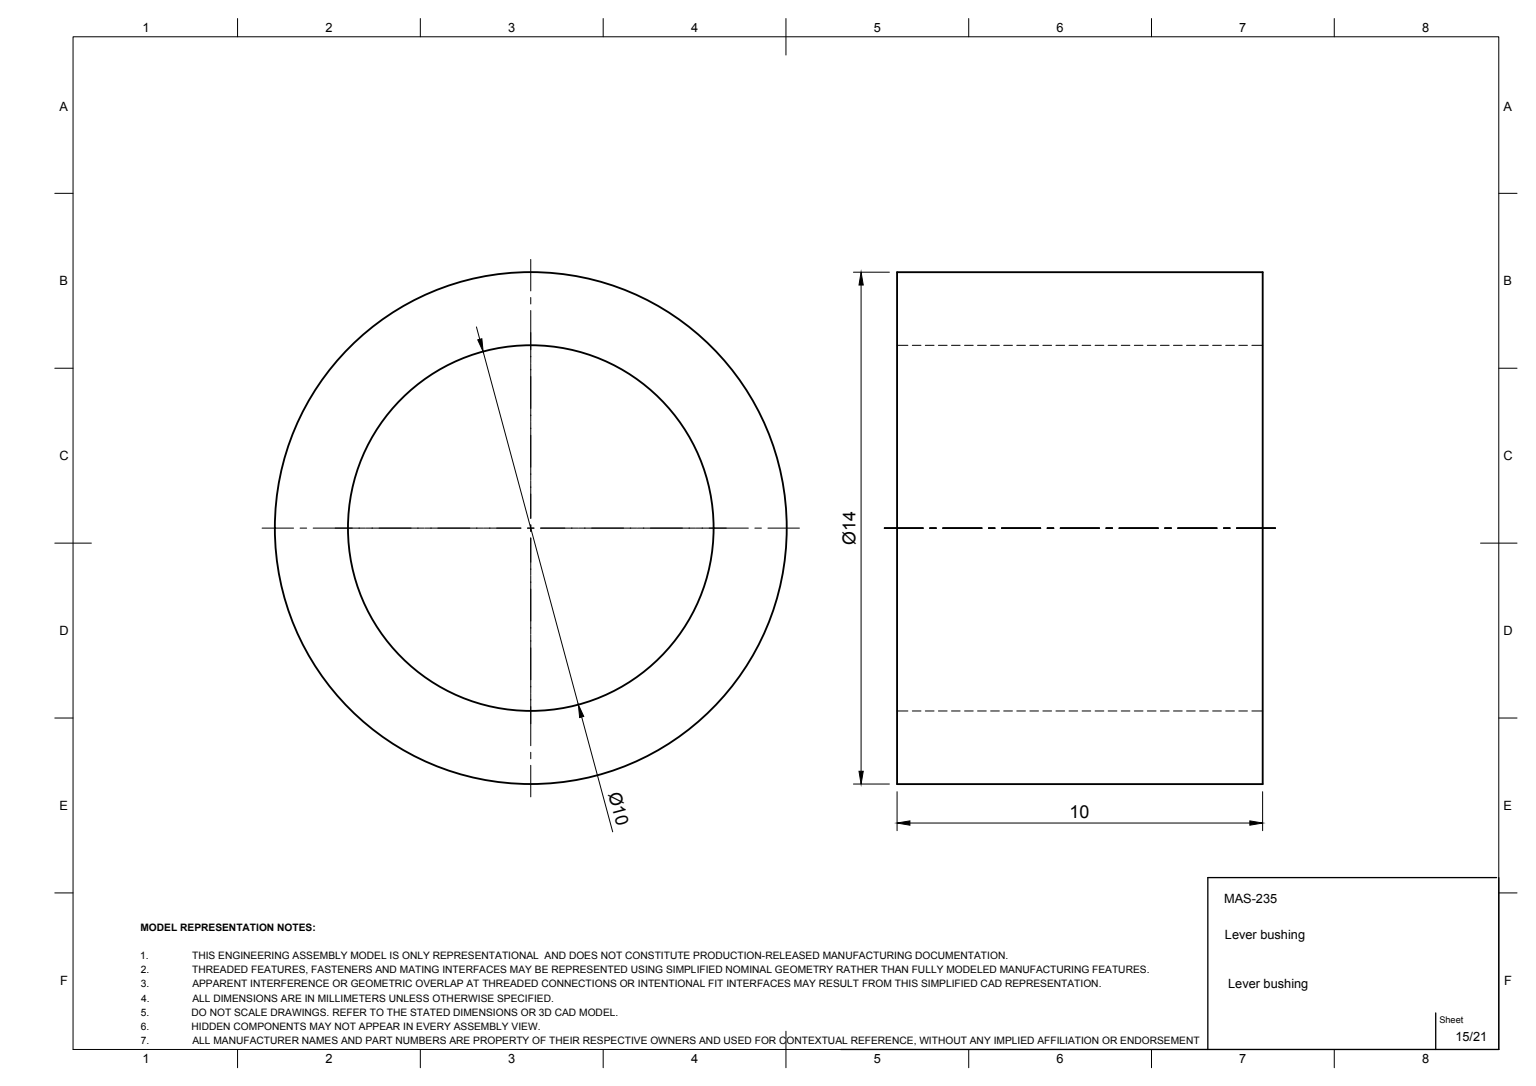
ISO-10303-21;
HEADER;
/* Generated by software containing ST-Developer
 * from STEP Tools, Inc. (www.steptools.com) 
 */

FILE_DESCRIPTION(
/* description */ ('Independent Whitworth quick-return mechanism. Crank radius40, ground-
center spacing80, lever180, connecting rod160, output guide X200. Nomi
nal stroke180 and long/short phase ratio2. Retained guide rods, replac
eable bearing sleeves and captured sliding shoe. No load or production
 rating assigned.'),
/* implementation_level */ '2;1');

FILE_NAME(
/* name */ 'Lever bushing.step',
/* time_stamp */ '2026-11-09T18:22:56-08:00',
/* author */ (''),
/* organization */ (''),
/* preprocessor_version */ 'ST-DEVELOPER v20.2',
/* originating_system */ 'Autodesk Translation Framework v15.17.0.0',
/* authorisation */ '');

FILE_SCHEMA (('AUTOMOTIVE_DESIGN { 1 0 10303 214 3 1 1 }'));
ENDSEC;

DATA;
#10=MECHANICAL_DESIGN_GEOMETRIC_PRESENTATION_REPRESENTATION('',(#236),#4388);
#196=SHAPE_REPRESENTATION_RELATIONSHIP('SRR','None',#4495,#216);
#216=ADVANCED_BREP_SHAPE_REPRESENTATION('',(#256),#4385);
#236=STYLED_ITEM('',(#4597),#256);
#256=MANIFOLD_SOLID_BREP('Body1',#2341);
#315=FACE_BOUND('',#744,.T.);
#316=FACE_BOUND('',#746,.T.);
#397=PLANE('',#2833);
#398=PLANE('',#2834);
#538=FACE_OUTER_BOUND('',#741,.T.);
#539=FACE_OUTER_BOUND('',#742,.T.);
#540=FACE_OUTER_BOUND('',#743,.T.);
#541=FACE_OUTER_BOUND('',#745,.T.);
#741=EDGE_LOOP('',(#2068,#2069,#2070,#2071));
#742=EDGE_LOOP('',(#2072,#2073,#2074,#2075));
#743=EDGE_LOOP('',(#2076));
#744=EDGE_LOOP('',(#2077));
#745=EDGE_LOOP('',(#2078));
#746=EDGE_LOOP('',(#2079));
#886=LINE('',#4251,#1025);
#887=LINE('',#4257,#1026);
#1025=VECTOR('',#3552,5.);
#1026=VECTOR('',#3559,7.);
#1147=CIRCLE('',#2828,5.);
#1148=CIRCLE('',#2829,5.);
#1149=CIRCLE('',#2831,7.);
#1150=CIRCLE('',#2832,7.);
#1317=VERTEX_POINT('',#4248);
#1318=VERTEX_POINT('',#4250);
#1319=VERTEX_POINT('',#4254);
#1320=VERTEX_POINT('',#4256);
#1570=EDGE_CURVE('',#1317,#1317,#1147,.T.);
#1571=EDGE_CURVE('',#1317,#1318,#886,.T.);
#1572=EDGE_CURVE('',#1318,#1318,#1148,.T.);
#1573=EDGE_CURVE('',#1319,#1319,#1149,.T.);
#1574=EDGE_CURVE('',#1319,#1320,#887,.T.);
#1575=EDGE_CURVE('',#1320,#1320,#1150,.T.);
#2068=ORIENTED_EDGE('',*,*,#1570,.F.);
#2069=ORIENTED_EDGE('',*,*,#1571,.T.);
#2070=ORIENTED_EDGE('',*,*,#1572,.T.);
#2071=ORIENTED_EDGE('',*,*,#1571,.F.);
#2072=ORIENTED_EDGE('',*,*,#1573,.F.);
#2073=ORIENTED_EDGE('',*,*,#1574,.T.);
#2074=ORIENTED_EDGE('',*,*,#1575,.T.);
#2075=ORIENTED_EDGE('',*,*,#1574,.F.);
#2076=ORIENTED_EDGE('',*,*,#1573,.T.);
#2077=ORIENTED_EDGE('',*,*,#1570,.T.);
#2078=ORIENTED_EDGE('',*,*,#1575,.F.);
#2079=ORIENTED_EDGE('',*,*,#1572,.F.);
#2171=CYLINDRICAL_SURFACE('',#2827,5.);
#2172=CYLINDRICAL_SURFACE('',#2830,7.);
#2310=ADVANCED_FACE('',(#538),#2171,.F.);
#2311=ADVANCED_FACE('',(#539),#2172,.T.);
#2312=ADVANCED_FACE('',(#540,#315),#397,.T.);
#2313=ADVANCED_FACE('',(#541,#316),#398,.F.);
#2341=CLOSED_SHELL('',(#2310,#2311,#2312,#2313));
#2826=AXIS2_PLACEMENT_3D('',#4246,#3546,#3547);
#2827=AXIS2_PLACEMENT_3D('',#4247,#3548,#3549);
#2828=AXIS2_PLACEMENT_3D('',#4249,#3550,#3551);
#2829=AXIS2_PLACEMENT_3D('',#4252,#3553,#3554);
#2830=AXIS2_PLACEMENT_3D('',#4253,#3555,#3556);
#2831=AXIS2_PLACEMENT_3D('',#4255,#3557,#3558);
#2832=AXIS2_PLACEMENT_3D('',#4258,#3560,#3561);
#2833=AXIS2_PLACEMENT_3D('',#4259,#3562,#3563);
#2834=AXIS2_PLACEMENT_3D('',#4260,#3564,#3565);
#3546=DIRECTION('axis',(0.,0.,1.));
#3547=DIRECTION('refdir',(1.,0.,0.));
#3548=DIRECTION('center_axis',(0.,0.,1.));
#3549=DIRECTION('ref_axis',(1.,0.,0.));
#3550=DIRECTION('center_axis',(0.,0.,-1.));
#3551=DIRECTION('ref_axis',(1.,0.,0.));
#3552=DIRECTION('',(0.,0.,-1.));
#3553=DIRECTION('center_axis',(0.,0.,-1.));
#3554=DIRECTION('ref_axis',(1.,0.,0.));
#3555=DIRECTION('center_axis',(0.,0.,1.));
#3556=DIRECTION('ref_axis',(1.,0.,0.));
#3557=DIRECTION('center_axis',(0.,0.,1.));
#3558=DIRECTION('ref_axis',(1.,0.,0.));
#3559=DIRECTION('',(0.,0.,-1.));
#3560=DIRECTION('center_axis',(0.,0.,1.));
#3561=DIRECTION('ref_axis',(1.,0.,0.));
#3562=DIRECTION('center_axis',(0.,0.,1.));
#3563=DIRECTION('ref_axis',(1.,0.,0.));
#3564=DIRECTION('center_axis',(0.,0.,1.));
#3565=DIRECTION('ref_axis',(1.,0.,0.));
#4246=CARTESIAN_POINT('',(0.,0.,0.));
#4247=CARTESIAN_POINT('Origin',(0.,0.,0.));
#4248=CARTESIAN_POINT('',(-5.,-6.12323399573677E-16,10.));
#4249=CARTESIAN_POINT('Origin',(0.,0.,10.));
#4250=CARTESIAN_POINT('',(-5.,-6.12323399573677E-16,0.));
#4251=CARTESIAN_POINT('',(-5.,-6.12323399573677E-16,0.));
#4252=CARTESIAN_POINT('Origin',(0.,0.,0.));
#4253=CARTESIAN_POINT('Origin',(0.,0.,0.));
#4254=CARTESIAN_POINT('',(-7.,-8.57252759403147E-16,10.));
#4255=CARTESIAN_POINT('Origin',(0.,0.,10.));
#4256=CARTESIAN_POINT('',(-7.,-8.57252759403147E-16,0.));
#4257=CARTESIAN_POINT('',(-7.,-8.57252759403147E-16,0.));
#4258=CARTESIAN_POINT('Origin',(0.,0.,0.));
#4259=CARTESIAN_POINT('Origin',(0.,0.,10.));
#4260=CARTESIAN_POINT('Origin',(0.,0.,0.));
#4363=UNCERTAINTY_MEASURE_WITH_UNIT(LENGTH_MEASURE(0.01),#4389,
'DISTANCE_ACCURACY_VALUE',
'Maximum model space distance between geometric entities at asserted c
onnectivities');
#4366=UNCERTAINTY_MEASURE_WITH_UNIT(LENGTH_MEASURE(0.01),#4389,
'DISTANCE_ACCURACY_VALUE',
'Maximum model space distance between geometric entities at asserted c
onnectivities');
#4385=(
GEOMETRIC_REPRESENTATION_CONTEXT(3)
GLOBAL_UNCERTAINTY_ASSIGNED_CONTEXT((#4363))
GLOBAL_UNIT_ASSIGNED_CONTEXT((#4389,#4391,#4392))
REPRESENTATION_CONTEXT('','3D')
);
#4388=(
GEOMETRIC_REPRESENTATION_CONTEXT(3)
GLOBAL_UNCERTAINTY_ASSIGNED_CONTEXT((#4366))
GLOBAL_UNIT_ASSIGNED_CONTEXT((#4389,#4391,#4392))
REPRESENTATION_CONTEXT('','3D')
);
#4389=(
LENGTH_UNIT()
NAMED_UNIT(*)
SI_UNIT(.MILLI.,.METRE.)
);
#4391=(
NAMED_UNIT(*)
PLANE_ANGLE_UNIT()
SI_UNIT($,.RADIAN.)
);
#4392=(
NAMED_UNIT(*)
SI_UNIT($,.STERADIAN.)
SOLID_ANGLE_UNIT()
);
#4411=SHAPE_DEFINITION_REPRESENTATION(#4432,#4495);
#4432=PRODUCT_DEFINITION_SHAPE('',$,#4517);
#4495=SHAPE_REPRESENTATION('',(#2826),#4385);
#4498=PRODUCT_DEFINITION_CONTEXT('part definition',#4563,'design');
#4517=PRODUCT_DEFINITION('Lever bushing','Lever bushing',#4538,#4498);
#4538=PRODUCT_DEFINITION_FORMATION('',$,#4583);
#4563=APPLICATION_CONTEXT(
'Core Data for Automotive Mechanical Design Process');
#4564=PRODUCT_CONTEXT('part definition',#4563,'mechanical');
#4583=PRODUCT('Lever bushing','Lever bushing',$,(#4564));
#4597=PRESENTATION_STYLE_ASSIGNMENT((#4611));
#4611=SURFACE_STYLE_USAGE(.BOTH.,#4625);
#4625=SURFACE_SIDE_STYLE('',(#4639));
#4639=SURFACE_STYLE_FILL_AREA(#4653);
#4653=FILL_AREA_STYLE('Bearing gray',(#4667));
#4667=FILL_AREA_STYLE_COLOUR('Bearing gray',#4681);
#4681=COLOUR_RGB('Bearing gray',0.725490196078431,0.752941176470588,0.792156862745098);
ENDSEC;
END-ISO-10303-21;
